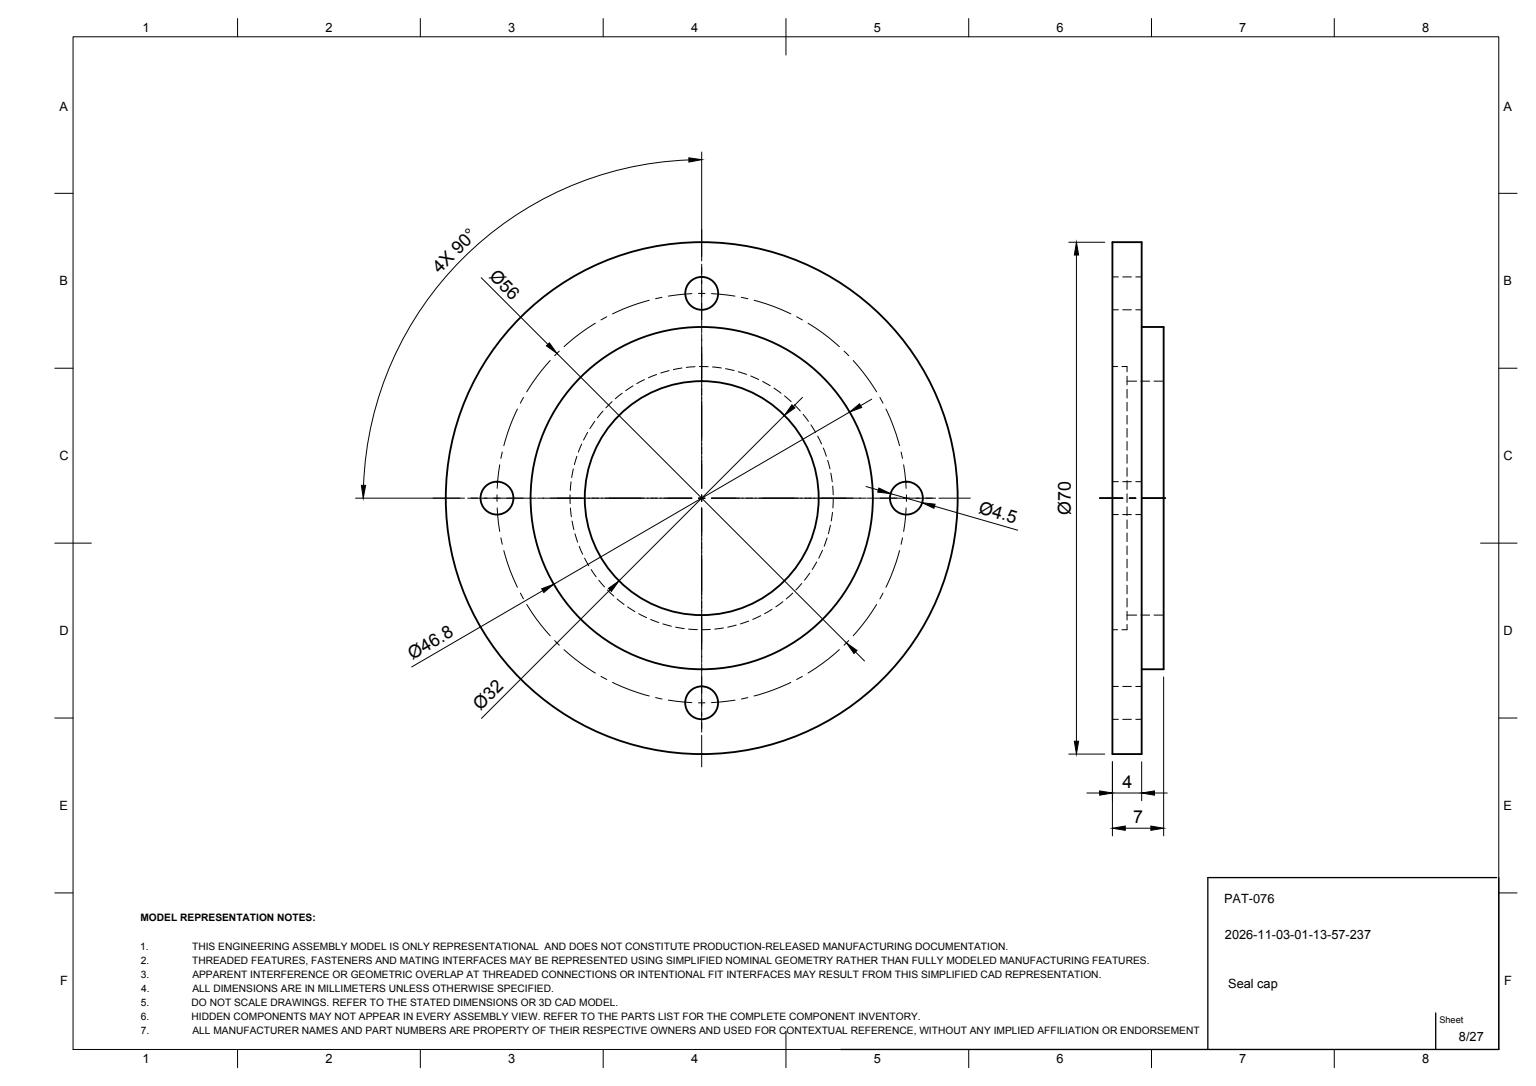
ISO-10303-21;
HEADER;
/* Generated by software containing ST-Developer
 * from STEP Tools, Inc. (www.steptools.com) 
 */

FILE_DESCRIPTION(
/* description */ ('Overhung pulley bearing cartridge'),
/* implementation_level */ '2;1');

FILE_NAME(
/* name */ 'Seal cap.step',
/* time_stamp */ '2026-10-28T03:22:33-07:00',
/* author */ (''),
/* organization */ (''),
/* preprocessor_version */ 'ST-DEVELOPER v20.2',
/* originating_system */ 'Autodesk Translation Framework v15.17.0.0',
/* authorisation */ '');

FILE_SCHEMA (('AUTOMOTIVE_DESIGN { 1 0 10303 214 3 1 1 }'));
ENDSEC;

DATA;
#10=MECHANICAL_DESIGN_GEOMETRIC_PRESENTATION_REPRESENTATION('',(#286),#10963);
#242=SHAPE_REPRESENTATION_RELATIONSHIP('SRR','None',#11062,#264);
#264=ADVANCED_BREP_SHAPE_REPRESENTATION('',(#316),#10942);
#286=STYLED_ITEM('',(#11260),#316);
#316=MANIFOLD_SOLID_BREP('Body1',#5653);
#371=FACE_BOUND('',#998,.T.);
#372=FACE_BOUND('',#1001,.T.);
#373=FACE_BOUND('',#1005,.T.);
#374=FACE_BOUND('',#1006,.T.);
#375=FACE_BOUND('',#1007,.T.);
#376=FACE_BOUND('',#1008,.T.);
#377=FACE_BOUND('',#1009,.T.);
#378=FACE_BOUND('',#1011,.T.);
#379=FACE_BOUND('',#1012,.T.);
#380=FACE_BOUND('',#1013,.T.);
#381=FACE_BOUND('',#1014,.T.);
#382=FACE_BOUND('',#1015,.T.);
#470=PLANE('',#6050);
#471=PLANE('',#6055);
#472=PLANE('',#6061);
#473=PLANE('',#6062);
#633=FACE_OUTER_BOUND('',#992,.T.);
#634=FACE_OUTER_BOUND('',#993,.T.);
#635=FACE_OUTER_BOUND('',#994,.T.);
#636=FACE_OUTER_BOUND('',#995,.T.);
#637=FACE_OUTER_BOUND('',#996,.T.);
#638=FACE_OUTER_BOUND('',#997,.T.);
#639=FACE_OUTER_BOUND('',#999,.T.);
#640=FACE_OUTER_BOUND('',#1000,.T.);
#641=FACE_OUTER_BOUND('',#1002,.T.);
#642=FACE_OUTER_BOUND('',#1003,.T.);
#643=FACE_OUTER_BOUND('',#1004,.T.);
#644=FACE_OUTER_BOUND('',#1010,.T.);
#992=EDGE_LOOP('',(#3885,#3886,#3887,#3888));
#993=EDGE_LOOP('',(#3889,#3890,#3891,#3892));
#994=EDGE_LOOP('',(#3893,#3894,#3895,#3896));
#995=EDGE_LOOP('',(#3897,#3898,#3899,#3900));
#996=EDGE_LOOP('',(#3901,#3902,#3903,#3904));
#997=EDGE_LOOP('',(#3905));
#998=EDGE_LOOP('',(#3906));
#999=EDGE_LOOP('',(#3907,#3908,#3909,#3910));
#1000=EDGE_LOOP('',(#3911));
#1001=EDGE_LOOP('',(#3912));
#1002=EDGE_LOOP('',(#3913,#3914,#3915,#3916));
#1003=EDGE_LOOP('',(#3917,#3918,#3919,#3920));
#1004=EDGE_LOOP('',(#3921));
#1005=EDGE_LOOP('',(#3922));
#1006=EDGE_LOOP('',(#3923));
#1007=EDGE_LOOP('',(#3924));
#1008=EDGE_LOOP('',(#3925));
#1009=EDGE_LOOP('',(#3926));
#1010=EDGE_LOOP('',(#3927));
#1011=EDGE_LOOP('',(#3928));
#1012=EDGE_LOOP('',(#3929));
#1013=EDGE_LOOP('',(#3930));
#1014=EDGE_LOOP('',(#3931));
#1015=EDGE_LOOP('',(#3932));
#1396=LINE('',#8814,#1738);
#1397=LINE('',#8820,#1739);
#1398=LINE('',#8826,#1740);
#1399=LINE('',#8832,#1741);
#1400=LINE('',#8838,#1742);
#1401=LINE('',#8847,#1743);
#1402=LINE('',#8853,#1744);
#1403=LINE('',#8858,#1745);
#1738=VECTOR('',#6980,0.225);
#1739=VECTOR('',#6987,0.225);
#1740=VECTOR('',#6994,0.225);
#1741=VECTOR('',#7001,0.225);
#1742=VECTOR('',#7008,2.34);
#1743=VECTOR('',#7019,1.8);
#1744=VECTOR('',#7028,1.6);
#1745=VECTOR('',#7033,3.5);
#2060=CIRCLE('',#6036,0.225);
#2061=CIRCLE('',#6037,0.225);
#2062=CIRCLE('',#6039,0.225);
#2063=CIRCLE('',#6040,0.225);
#2064=CIRCLE('',#6042,0.225);
#2065=CIRCLE('',#6043,0.225);
#2066=CIRCLE('',#6045,0.225);
#2067=CIRCLE('',#6046,0.225);
#2068=CIRCLE('',#6048,2.34);
#2069=CIRCLE('',#6049,2.34);
#2070=CIRCLE('',#6051,1.6);
#2071=CIRCLE('',#6053,1.8);
#2072=CIRCLE('',#6054,1.8);
#2073=CIRCLE('',#6056,1.6);
#2074=CIRCLE('',#6059,3.5);
#2075=CIRCLE('',#6060,3.5);
#2459=VERTEX_POINT('',#8811);
#2460=VERTEX_POINT('',#8813);
#2461=VERTEX_POINT('',#8817);
#2462=VERTEX_POINT('',#8819);
#2463=VERTEX_POINT('',#8823);
#2464=VERTEX_POINT('',#8825);
#2465=VERTEX_POINT('',#8829);
#2466=VERTEX_POINT('',#8831);
#2467=VERTEX_POINT('',#8835);
#2468=VERTEX_POINT('',#8837);
#2469=VERTEX_POINT('',#8841);
#2470=VERTEX_POINT('',#8844);
#2471=VERTEX_POINT('',#8846);
#2472=VERTEX_POINT('',#8850);
#2473=VERTEX_POINT('',#8855);
#2474=VERTEX_POINT('',#8857);
#3012=EDGE_CURVE('',#2459,#2459,#2060,.T.);
#3013=EDGE_CURVE('',#2459,#2460,#1396,.T.);
#3014=EDGE_CURVE('',#2460,#2460,#2061,.T.);
#3015=EDGE_CURVE('',#2461,#2461,#2062,.T.);
#3016=EDGE_CURVE('',#2461,#2462,#1397,.T.);
#3017=EDGE_CURVE('',#2462,#2462,#2063,.T.);
#3018=EDGE_CURVE('',#2463,#2463,#2064,.T.);
#3019=EDGE_CURVE('',#2463,#2464,#1398,.T.);
#3020=EDGE_CURVE('',#2464,#2464,#2065,.T.);
#3021=EDGE_CURVE('',#2465,#2465,#2066,.T.);
#3022=EDGE_CURVE('',#2465,#2466,#1399,.T.);
#3023=EDGE_CURVE('',#2466,#2466,#2067,.T.);
#3024=EDGE_CURVE('',#2467,#2467,#2068,.T.);
#3025=EDGE_CURVE('',#2467,#2468,#1400,.T.);
#3026=EDGE_CURVE('',#2468,#2468,#2069,.T.);
#3027=EDGE_CURVE('',#2469,#2469,#2070,.T.);
#3028=EDGE_CURVE('',#2470,#2470,#2071,.T.);
#3029=EDGE_CURVE('',#2470,#2471,#1401,.T.);
#3030=EDGE_CURVE('',#2471,#2471,#2072,.T.);
#3031=EDGE_CURVE('',#2472,#2472,#2073,.T.);
#3032=EDGE_CURVE('',#2469,#2472,#1402,.T.);
#3033=EDGE_CURVE('',#2473,#2473,#2074,.T.);
#3034=EDGE_CURVE('',#2473,#2474,#1403,.T.);
#3035=EDGE_CURVE('',#2474,#2474,#2075,.T.);
#3885=ORIENTED_EDGE('',*,*,#3012,.F.);
#3886=ORIENTED_EDGE('',*,*,#3013,.T.);
#3887=ORIENTED_EDGE('',*,*,#3014,.F.);
#3888=ORIENTED_EDGE('',*,*,#3013,.F.);
#3889=ORIENTED_EDGE('',*,*,#3015,.F.);
#3890=ORIENTED_EDGE('',*,*,#3016,.T.);
#3891=ORIENTED_EDGE('',*,*,#3017,.F.);
#3892=ORIENTED_EDGE('',*,*,#3016,.F.);
#3893=ORIENTED_EDGE('',*,*,#3018,.F.);
#3894=ORIENTED_EDGE('',*,*,#3019,.T.);
#3895=ORIENTED_EDGE('',*,*,#3020,.F.);
#3896=ORIENTED_EDGE('',*,*,#3019,.F.);
#3897=ORIENTED_EDGE('',*,*,#3021,.F.);
#3898=ORIENTED_EDGE('',*,*,#3022,.T.);
#3899=ORIENTED_EDGE('',*,*,#3023,.F.);
#3900=ORIENTED_EDGE('',*,*,#3022,.F.);
#3901=ORIENTED_EDGE('',*,*,#3024,.F.);
#3902=ORIENTED_EDGE('',*,*,#3025,.T.);
#3903=ORIENTED_EDGE('',*,*,#3026,.F.);
#3904=ORIENTED_EDGE('',*,*,#3025,.F.);
#3905=ORIENTED_EDGE('',*,*,#3024,.T.);
#3906=ORIENTED_EDGE('',*,*,#3027,.T.);
#3907=ORIENTED_EDGE('',*,*,#3028,.F.);
#3908=ORIENTED_EDGE('',*,*,#3029,.T.);
#3909=ORIENTED_EDGE('',*,*,#3030,.T.);
#3910=ORIENTED_EDGE('',*,*,#3029,.F.);
#3911=ORIENTED_EDGE('',*,*,#3030,.F.);
#3912=ORIENTED_EDGE('',*,*,#3031,.F.);
#3913=ORIENTED_EDGE('',*,*,#3027,.F.);
#3914=ORIENTED_EDGE('',*,*,#3032,.T.);
#3915=ORIENTED_EDGE('',*,*,#3031,.T.);
#3916=ORIENTED_EDGE('',*,*,#3032,.F.);
#3917=ORIENTED_EDGE('',*,*,#3033,.F.);
#3918=ORIENTED_EDGE('',*,*,#3034,.T.);
#3919=ORIENTED_EDGE('',*,*,#3035,.T.);
#3920=ORIENTED_EDGE('',*,*,#3034,.F.);
#3921=ORIENTED_EDGE('',*,*,#3033,.T.);
#3922=ORIENTED_EDGE('',*,*,#3026,.T.);
#3923=ORIENTED_EDGE('',*,*,#3023,.T.);
#3924=ORIENTED_EDGE('',*,*,#3020,.T.);
#3925=ORIENTED_EDGE('',*,*,#3017,.T.);
#3926=ORIENTED_EDGE('',*,*,#3014,.T.);
#3927=ORIENTED_EDGE('',*,*,#3035,.F.);
#3928=ORIENTED_EDGE('',*,*,#3028,.T.);
#3929=ORIENTED_EDGE('',*,*,#3021,.T.);
#3930=ORIENTED_EDGE('',*,*,#3018,.T.);
#3931=ORIENTED_EDGE('',*,*,#3015,.T.);
#3932=ORIENTED_EDGE('',*,*,#3012,.T.);
#5187=CYLINDRICAL_SURFACE('',#6035,0.225);
#5188=CYLINDRICAL_SURFACE('',#6038,0.225);
#5189=CYLINDRICAL_SURFACE('',#6041,0.225);
#5190=CYLINDRICAL_SURFACE('',#6044,0.225);
#5191=CYLINDRICAL_SURFACE('',#6047,2.34);
#5192=CYLINDRICAL_SURFACE('',#6052,1.8);
#5193=CYLINDRICAL_SURFACE('',#6057,1.6);
#5194=CYLINDRICAL_SURFACE('',#6058,3.5);
#5377=ADVANCED_FACE('',(#633),#5187,.F.);
#5378=ADVANCED_FACE('',(#634),#5188,.F.);
#5379=ADVANCED_FACE('',(#635),#5189,.F.);
#5380=ADVANCED_FACE('',(#636),#5190,.F.);
#5381=ADVANCED_FACE('',(#637),#5191,.T.);
#5382=ADVANCED_FACE('',(#638,#371),#470,.T.);
#5383=ADVANCED_FACE('',(#639),#5192,.F.);
#5384=ADVANCED_FACE('',(#640,#372),#471,.F.);
#5385=ADVANCED_FACE('',(#641),#5193,.F.);
#5386=ADVANCED_FACE('',(#642),#5194,.T.);
#5387=ADVANCED_FACE('',(#643,#373,#374,#375,#376,#377),#472,.T.);
#5388=ADVANCED_FACE('',(#644,#378,#379,#380,#381,#382),#473,.F.);
#5653=CLOSED_SHELL('',(#5377,#5378,#5379,#5380,#5381,#5382,#5383,#5384,
#5385,#5386,#5387,#5388));
#6034=AXIS2_PLACEMENT_3D('',#8809,#6974,#6975);
#6035=AXIS2_PLACEMENT_3D('',#8810,#6976,#6977);
#6036=AXIS2_PLACEMENT_3D('',#8812,#6978,#6979);
#6037=AXIS2_PLACEMENT_3D('',#8815,#6981,#6982);
#6038=AXIS2_PLACEMENT_3D('',#8816,#6983,#6984);
#6039=AXIS2_PLACEMENT_3D('',#8818,#6985,#6986);
#6040=AXIS2_PLACEMENT_3D('',#8821,#6988,#6989);
#6041=AXIS2_PLACEMENT_3D('',#8822,#6990,#6991);
#6042=AXIS2_PLACEMENT_3D('',#8824,#6992,#6993);
#6043=AXIS2_PLACEMENT_3D('',#8827,#6995,#6996);
#6044=AXIS2_PLACEMENT_3D('',#8828,#6997,#6998);
#6045=AXIS2_PLACEMENT_3D('',#8830,#6999,#7000);
#6046=AXIS2_PLACEMENT_3D('',#8833,#7002,#7003);
#6047=AXIS2_PLACEMENT_3D('',#8834,#7004,#7005);
#6048=AXIS2_PLACEMENT_3D('',#8836,#7006,#7007);
#6049=AXIS2_PLACEMENT_3D('',#8839,#7009,#7010);
#6050=AXIS2_PLACEMENT_3D('',#8840,#7011,#7012);
#6051=AXIS2_PLACEMENT_3D('',#8842,#7013,#7014);
#6052=AXIS2_PLACEMENT_3D('',#8843,#7015,#7016);
#6053=AXIS2_PLACEMENT_3D('',#8845,#7017,#7018);
#6054=AXIS2_PLACEMENT_3D('',#8848,#7020,#7021);
#6055=AXIS2_PLACEMENT_3D('',#8849,#7022,#7023);
#6056=AXIS2_PLACEMENT_3D('',#8851,#7024,#7025);
#6057=AXIS2_PLACEMENT_3D('',#8852,#7026,#7027);
#6058=AXIS2_PLACEMENT_3D('',#8854,#7029,#7030);
#6059=AXIS2_PLACEMENT_3D('',#8856,#7031,#7032);
#6060=AXIS2_PLACEMENT_3D('',#8859,#7034,#7035);
#6061=AXIS2_PLACEMENT_3D('',#8860,#7036,#7037);
#6062=AXIS2_PLACEMENT_3D('',#8861,#7038,#7039);
#6974=DIRECTION('axis',(0.,0.,1.));
#6975=DIRECTION('refdir',(1.,0.,0.));
#6976=DIRECTION('center_axis',(0.,1.,0.));
#6977=DIRECTION('ref_axis',(1.,0.,0.));
#6978=DIRECTION('center_axis',(0.,1.,0.));
#6979=DIRECTION('ref_axis',(1.,0.,0.));
#6980=DIRECTION('',(0.,1.,0.));
#6981=DIRECTION('center_axis',(0.,-1.,0.));
#6982=DIRECTION('ref_axis',(1.,0.,0.));
#6983=DIRECTION('center_axis',(0.,1.,0.));
#6984=DIRECTION('ref_axis',(1.,0.,0.));
#6985=DIRECTION('center_axis',(0.,1.,0.));
#6986=DIRECTION('ref_axis',(1.,0.,0.));
#6987=DIRECTION('',(0.,1.,0.));
#6988=DIRECTION('center_axis',(0.,-1.,0.));
#6989=DIRECTION('ref_axis',(1.,0.,0.));
#6990=DIRECTION('center_axis',(0.,1.,0.));
#6991=DIRECTION('ref_axis',(1.,0.,0.));
#6992=DIRECTION('center_axis',(0.,1.,0.));
#6993=DIRECTION('ref_axis',(1.,0.,0.));
#6994=DIRECTION('',(0.,1.,0.));
#6995=DIRECTION('center_axis',(0.,-1.,0.));
#6996=DIRECTION('ref_axis',(1.,0.,0.));
#6997=DIRECTION('center_axis',(0.,1.,0.));
#6998=DIRECTION('ref_axis',(1.,0.,0.));
#6999=DIRECTION('center_axis',(0.,1.,0.));
#7000=DIRECTION('ref_axis',(1.,0.,0.));
#7001=DIRECTION('',(0.,1.,0.));
#7002=DIRECTION('center_axis',(0.,-1.,0.));
#7003=DIRECTION('ref_axis',(1.,0.,0.));
#7004=DIRECTION('center_axis',(0.,1.,0.));
#7005=DIRECTION('ref_axis',(1.,0.,0.));
#7006=DIRECTION('center_axis',(0.,1.,0.));
#7007=DIRECTION('ref_axis',(1.,0.,0.));
#7008=DIRECTION('',(0.,-1.,0.));
#7009=DIRECTION('center_axis',(0.,-1.,0.));
#7010=DIRECTION('ref_axis',(1.,0.,0.));
#7011=DIRECTION('center_axis',(0.,1.,0.));
#7012=DIRECTION('ref_axis',(1.,0.,0.));
#7013=DIRECTION('center_axis',(0.,-1.,0.));
#7014=DIRECTION('ref_axis',(1.,0.,0.));
#7015=DIRECTION('center_axis',(0.,1.,0.));
#7016=DIRECTION('ref_axis',(1.,0.,0.));
#7017=DIRECTION('center_axis',(0.,1.,0.));
#7018=DIRECTION('ref_axis',(1.,0.,0.));
#7019=DIRECTION('',(0.,1.,0.));
#7020=DIRECTION('center_axis',(0.,1.,0.));
#7021=DIRECTION('ref_axis',(1.,0.,0.));
#7022=DIRECTION('center_axis',(0.,1.,0.));
#7023=DIRECTION('ref_axis',(1.,0.,0.));
#7024=DIRECTION('center_axis',(0.,-1.,0.));
#7025=DIRECTION('ref_axis',(1.,0.,0.));
#7026=DIRECTION('center_axis',(0.,1.,0.));
#7027=DIRECTION('ref_axis',(1.,0.,0.));
#7028=DIRECTION('',(0.,-1.,0.));
#7029=DIRECTION('center_axis',(0.,1.,0.));
#7030=DIRECTION('ref_axis',(1.,0.,0.));
#7031=DIRECTION('center_axis',(0.,1.,0.));
#7032=DIRECTION('ref_axis',(1.,0.,0.));
#7033=DIRECTION('',(0.,-1.,0.));
#7034=DIRECTION('center_axis',(0.,1.,0.));
#7035=DIRECTION('ref_axis',(1.,0.,0.));
#7036=DIRECTION('center_axis',(0.,1.,0.));
#7037=DIRECTION('ref_axis',(1.,0.,0.));
#7038=DIRECTION('center_axis',(0.,1.,0.));
#7039=DIRECTION('ref_axis',(1.,0.,0.));
#8809=CARTESIAN_POINT('',(0.,0.,0.));
#8810=CARTESIAN_POINT('Origin',(-2.8,-0.5,4.5));
#8811=CARTESIAN_POINT('',(-3.025,-0.4,4.5));
#8812=CARTESIAN_POINT('Origin',(-2.8,-0.4,4.5));
#8813=CARTESIAN_POINT('',(-3.025,0.,4.5));
#8814=CARTESIAN_POINT('',(-3.025,-0.5,4.5));
#8815=CARTESIAN_POINT('Origin',(-2.8,0.,4.5));
#8816=CARTESIAN_POINT('Origin',(1.71450551880629E-16,-0.5,7.3));
#8817=CARTESIAN_POINT('',(-0.225,-0.4,7.3));
#8818=CARTESIAN_POINT('Origin',(1.71450551880629E-16,-0.4,7.3));
#8819=CARTESIAN_POINT('',(-0.225,0.,7.3));
#8820=CARTESIAN_POINT('',(-0.225,-0.5,7.3));
#8821=CARTESIAN_POINT('Origin',(1.71450551880629E-16,0.,7.3));
#8822=CARTESIAN_POINT('Origin',(2.8,-0.5,4.5));
#8823=CARTESIAN_POINT('',(2.575,-0.4,4.5));
#8824=CARTESIAN_POINT('Origin',(2.8,-0.4,4.5));
#8825=CARTESIAN_POINT('',(2.575,0.,4.5));
#8826=CARTESIAN_POINT('',(2.575,-0.5,4.5));
#8827=CARTESIAN_POINT('Origin',(2.8,0.,4.5));
#8828=CARTESIAN_POINT('Origin',(-5.14351655641888E-16,-0.5,1.7));
#8829=CARTESIAN_POINT('',(-0.225000000000001,-0.4,1.7));
#8830=CARTESIAN_POINT('Origin',(-5.14351655641888E-16,-0.4,1.7));
#8831=CARTESIAN_POINT('',(-0.225000000000001,0.,1.7));
#8832=CARTESIAN_POINT('',(-0.225000000000001,-0.5,1.7));
#8833=CARTESIAN_POINT('Origin',(-5.14351655641888E-16,0.,1.7));
#8834=CARTESIAN_POINT('Origin',(0.,0.,4.5));
#8835=CARTESIAN_POINT('',(-2.34,0.3,4.5));
#8836=CARTESIAN_POINT('Origin',(0.,0.3,4.5));
#8837=CARTESIAN_POINT('',(-2.34,0.,4.5));
#8838=CARTESIAN_POINT('',(-2.34,0.,4.5));
#8839=CARTESIAN_POINT('Origin',(0.,0.,4.5));
#8840=CARTESIAN_POINT('Origin',(0.,0.3,4.5));
#8841=CARTESIAN_POINT('',(-1.6,0.3,4.5));
#8842=CARTESIAN_POINT('Origin',(0.,0.3,4.5));
#8843=CARTESIAN_POINT('Origin',(0.,-0.41,4.5));
#8844=CARTESIAN_POINT('',(-1.8,-0.4,4.5));
#8845=CARTESIAN_POINT('Origin',(0.,-0.4,4.5));
#8846=CARTESIAN_POINT('',(-1.8,-0.2,4.5));
#8847=CARTESIAN_POINT('',(-1.8,-0.41,4.5));
#8848=CARTESIAN_POINT('Origin',(0.,-0.2,4.5));
#8849=CARTESIAN_POINT('Origin',(0.,-0.2,4.5));
#8850=CARTESIAN_POINT('',(-1.6,-0.2,4.5));
#8851=CARTESIAN_POINT('Origin',(0.,-0.2,4.5));
#8852=CARTESIAN_POINT('Origin',(0.,-0.4,4.5));
#8853=CARTESIAN_POINT('',(-1.6,-0.4,4.5));
#8854=CARTESIAN_POINT('Origin',(0.,-0.4,4.5));
#8855=CARTESIAN_POINT('',(-3.5,0.,4.5));
#8856=CARTESIAN_POINT('Origin',(0.,0.,4.5));
#8857=CARTESIAN_POINT('',(-3.5,-0.4,4.5));
#8858=CARTESIAN_POINT('',(-3.5,-0.4,4.5));
#8859=CARTESIAN_POINT('Origin',(0.,-0.4,4.5));
#8860=CARTESIAN_POINT('Origin',(0.,0.,4.5));
#8861=CARTESIAN_POINT('Origin',(0.,-0.4,4.5));
#10915=UNCERTAINTY_MEASURE_WITH_UNIT(LENGTH_MEASURE(0.001),#10964,
'DISTANCE_ACCURACY_VALUE',
'Maximum model space distance between geometric entities at asserted c
onnectivities');
#10936=UNCERTAINTY_MEASURE_WITH_UNIT(LENGTH_MEASURE(0.001),#10964,
'DISTANCE_ACCURACY_VALUE',
'Maximum model space distance between geometric entities at asserted c
onnectivities');
#10942=(
GEOMETRIC_REPRESENTATION_CONTEXT(3)
GLOBAL_UNCERTAINTY_ASSIGNED_CONTEXT((#10915))
GLOBAL_UNIT_ASSIGNED_CONTEXT((#10964,#10966,#10967))
REPRESENTATION_CONTEXT('','3D')
);
#10963=(
GEOMETRIC_REPRESENTATION_CONTEXT(3)
GLOBAL_UNCERTAINTY_ASSIGNED_CONTEXT((#10936))
GLOBAL_UNIT_ASSIGNED_CONTEXT((#10964,#10966,#10967))
REPRESENTATION_CONTEXT('','3D')
);
#10964=(
LENGTH_UNIT()
NAMED_UNIT(*)
SI_UNIT(.CENTI.,.METRE.)
);
#10966=(
NAMED_UNIT(*)
PLANE_ANGLE_UNIT()
SI_UNIT($,.RADIAN.)
);
#10967=(
NAMED_UNIT(*)
SI_UNIT($,.STERADIAN.)
SOLID_ANGLE_UNIT()
);
#10973=SHAPE_DEFINITION_REPRESENTATION(#10999,#11062);
#10999=PRODUCT_DEFINITION_SHAPE('',$,#11089);
#11062=SHAPE_REPRESENTATION('',(#6034),#10942);
#11083=PRODUCT_DEFINITION_CONTEXT('part definition',#11163,'design');
#11089=PRODUCT_DEFINITION('Seal cap','Seal cap',#11115,#11083);
#11115=PRODUCT_DEFINITION_FORMATION('',$,#11170);
#11163=APPLICATION_CONTEXT(
'Core Data for Automotive Mechanical Design Process');
#11164=PRODUCT_CONTEXT('part definition',#11163,'mechanical');
#11170=PRODUCT('Seal cap','Seal cap','Seal cap',(#11164));
#11254=COLOUR_RGB('Black',0.12,0.14,0.17);
#11255=FILL_AREA_STYLE_COLOUR('',#11254);
#11256=FILL_AREA_STYLE('',(#11255));
#11257=SURFACE_STYLE_FILL_AREA(#11256);
#11258=SURFACE_SIDE_STYLE('',(#11257));
#11259=SURFACE_STYLE_USAGE(.BOTH.,#11258);
#11260=PRESENTATION_STYLE_ASSIGNMENT((#11259));
ENDSEC;
END-ISO-10303-21;
